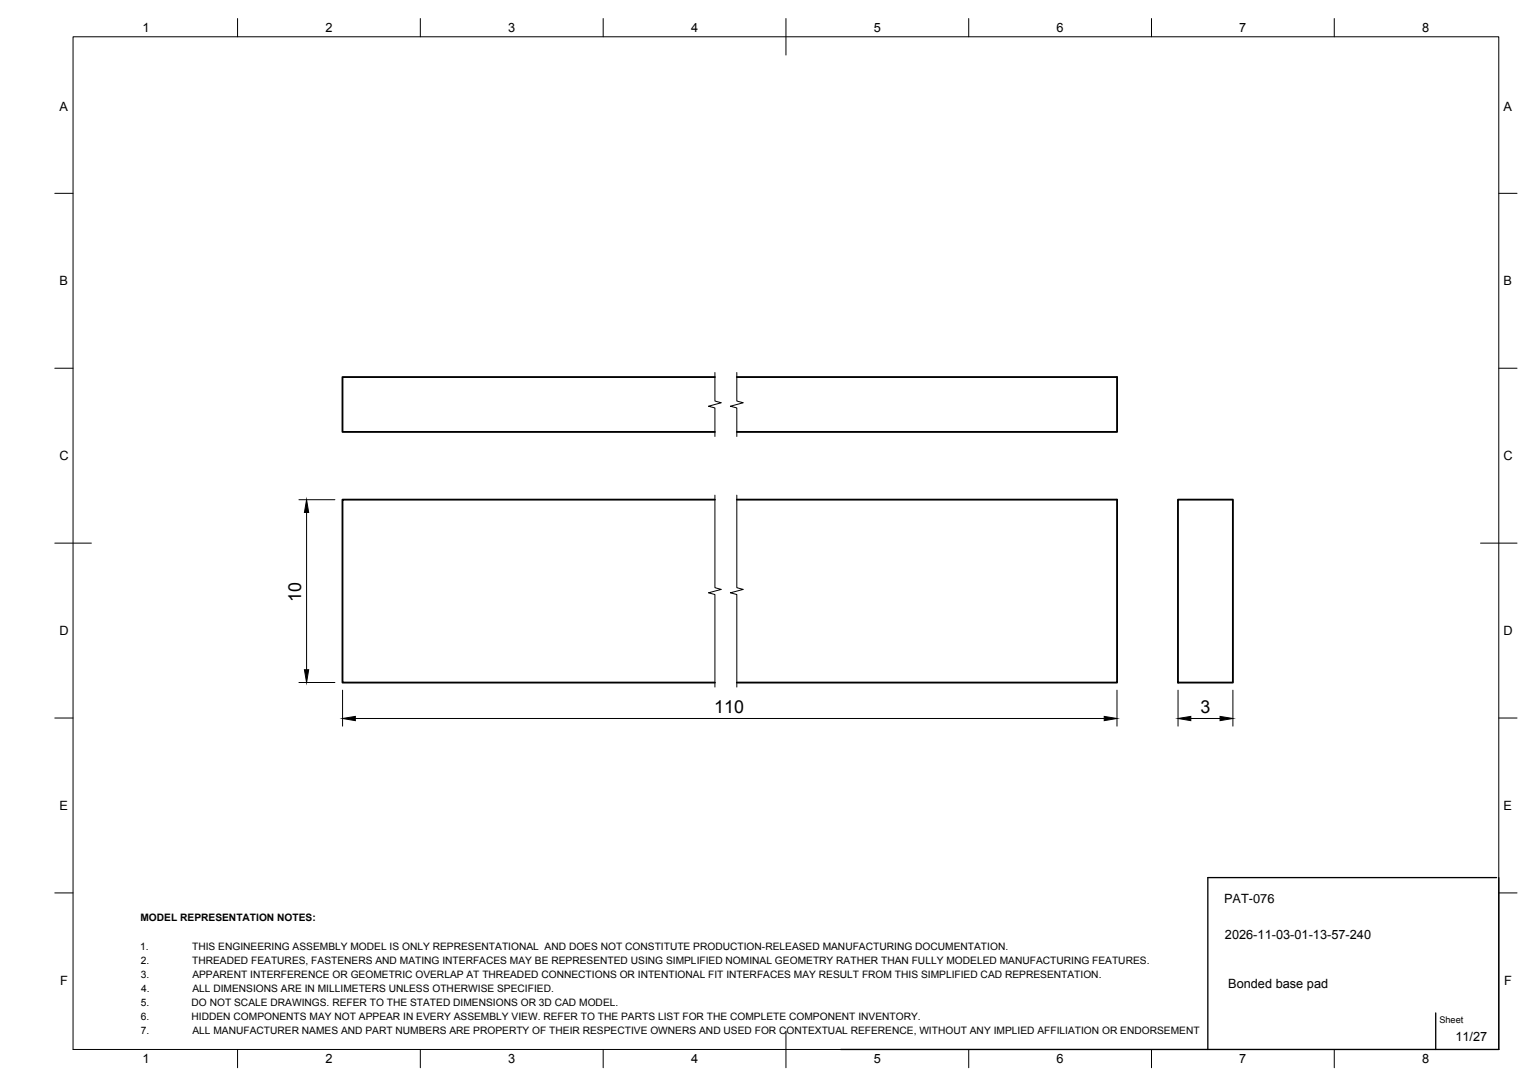
ISO-10303-21;
HEADER;
/* Generated by software containing ST-Developer
 * from STEP Tools, Inc. (www.steptools.com) 
 */

FILE_DESCRIPTION(
/* description */ ('Overhung pulley bearing cartridge'),
/* implementation_level */ '2;1');

FILE_NAME(
/* name */ 'Bonded base pad.step',
/* time_stamp */ '2026-10-28T03:22:33-07:00',
/* author */ (''),
/* organization */ (''),
/* preprocessor_version */ 'ST-DEVELOPER v20.2',
/* originating_system */ 'Autodesk Translation Framework v15.17.0.0',
/* authorisation */ '');

FILE_SCHEMA (('AUTOMOTIVE_DESIGN { 1 0 10303 214 3 1 1 }'));
ENDSEC;

DATA;
#10=MECHANICAL_DESIGN_GEOMETRIC_PRESENTATION_REPRESENTATION('',(#289),#10963);
#245=SHAPE_REPRESENTATION_RELATIONSHIP('SRR','None',#11065,#267);
#267=ADVANCED_BREP_SHAPE_REPRESENTATION('',(#319),#10945);
#289=STYLED_ITEM('',(#11232),#319);
#319=MANIFOLD_SOLID_BREP('Body1',#5656);
#479=PLANE('',#6098);
#480=PLANE('',#6099);
#481=PLANE('',#6100);
#482=PLANE('',#6101);
#483=PLANE('',#6102);
#484=PLANE('',#6103);
#659=FACE_OUTER_BOUND('',#1043,.T.);
#660=FACE_OUTER_BOUND('',#1044,.T.);
#661=FACE_OUTER_BOUND('',#1045,.T.);
#662=FACE_OUTER_BOUND('',#1046,.T.);
#663=FACE_OUTER_BOUND('',#1047,.T.);
#664=FACE_OUTER_BOUND('',#1048,.T.);
#1043=EDGE_LOOP('',(#3987,#3988,#3989,#3990));
#1044=EDGE_LOOP('',(#3991,#3992,#3993,#3994));
#1045=EDGE_LOOP('',(#3995,#3996,#3997,#3998));
#1046=EDGE_LOOP('',(#3999,#4000,#4001,#4002));
#1047=EDGE_LOOP('',(#4003,#4004,#4005,#4006));
#1048=EDGE_LOOP('',(#4007,#4008,#4009,#4010));
#1413=LINE('',#8927,#1755);
#1414=LINE('',#8929,#1756);
#1415=LINE('',#8931,#1757);
#1416=LINE('',#8932,#1758);
#1417=LINE('',#8935,#1759);
#1418=LINE('',#8937,#1760);
#1419=LINE('',#8938,#1761);
#1420=LINE('',#8941,#1762);
#1421=LINE('',#8943,#1763);
#1422=LINE('',#8944,#1764);
#1423=LINE('',#8946,#1765);
#1424=LINE('',#8947,#1766);
#1755=VECTOR('',#7121,1.);
#1756=VECTOR('',#7122,1.);
#1757=VECTOR('',#7123,1.);
#1758=VECTOR('',#7124,1.);
#1759=VECTOR('',#7127,1.);
#1760=VECTOR('',#7128,1.);
#1761=VECTOR('',#7129,1.);
#1762=VECTOR('',#7132,1.);
#1763=VECTOR('',#7133,1.);
#1764=VECTOR('',#7134,1.);
#1765=VECTOR('',#7137,1.);
#1766=VECTOR('',#7138,1.);
#2493=VERTEX_POINT('',#8925);
#2494=VERTEX_POINT('',#8926);
#2495=VERTEX_POINT('',#8928);
#2496=VERTEX_POINT('',#8930);
#2497=VERTEX_POINT('',#8934);
#2498=VERTEX_POINT('',#8936);
#2499=VERTEX_POINT('',#8940);
#2500=VERTEX_POINT('',#8942);
#3063=EDGE_CURVE('',#2493,#2494,#1413,.T.);
#3064=EDGE_CURVE('',#2494,#2495,#1414,.T.);
#3065=EDGE_CURVE('',#2496,#2495,#1415,.T.);
#3066=EDGE_CURVE('',#2493,#2496,#1416,.T.);
#3067=EDGE_CURVE('',#2497,#2493,#1417,.T.);
#3068=EDGE_CURVE('',#2498,#2496,#1418,.T.);
#3069=EDGE_CURVE('',#2497,#2498,#1419,.T.);
#3070=EDGE_CURVE('',#2499,#2497,#1420,.T.);
#3071=EDGE_CURVE('',#2500,#2498,#1421,.T.);
#3072=EDGE_CURVE('',#2499,#2500,#1422,.T.);
#3073=EDGE_CURVE('',#2494,#2499,#1423,.T.);
#3074=EDGE_CURVE('',#2495,#2500,#1424,.T.);
#3987=ORIENTED_EDGE('',*,*,#3063,.T.);
#3988=ORIENTED_EDGE('',*,*,#3064,.T.);
#3989=ORIENTED_EDGE('',*,*,#3065,.F.);
#3990=ORIENTED_EDGE('',*,*,#3066,.F.);
#3991=ORIENTED_EDGE('',*,*,#3067,.T.);
#3992=ORIENTED_EDGE('',*,*,#3066,.T.);
#3993=ORIENTED_EDGE('',*,*,#3068,.F.);
#3994=ORIENTED_EDGE('',*,*,#3069,.F.);
#3995=ORIENTED_EDGE('',*,*,#3070,.T.);
#3996=ORIENTED_EDGE('',*,*,#3069,.T.);
#3997=ORIENTED_EDGE('',*,*,#3071,.F.);
#3998=ORIENTED_EDGE('',*,*,#3072,.F.);
#3999=ORIENTED_EDGE('',*,*,#3073,.T.);
#4000=ORIENTED_EDGE('',*,*,#3072,.T.);
#4001=ORIENTED_EDGE('',*,*,#3074,.F.);
#4002=ORIENTED_EDGE('',*,*,#3064,.F.);
#4003=ORIENTED_EDGE('',*,*,#3074,.T.);
#4004=ORIENTED_EDGE('',*,*,#3071,.T.);
#4005=ORIENTED_EDGE('',*,*,#3068,.T.);
#4006=ORIENTED_EDGE('',*,*,#3065,.T.);
#4007=ORIENTED_EDGE('',*,*,#3073,.F.);
#4008=ORIENTED_EDGE('',*,*,#3063,.F.);
#4009=ORIENTED_EDGE('',*,*,#3067,.F.);
#4010=ORIENTED_EDGE('',*,*,#3070,.F.);
#5403=ADVANCED_FACE('',(#659),#479,.T.);
#5404=ADVANCED_FACE('',(#660),#480,.T.);
#5405=ADVANCED_FACE('',(#661),#481,.T.);
#5406=ADVANCED_FACE('',(#662),#482,.T.);
#5407=ADVANCED_FACE('',(#663),#483,.T.);
#5408=ADVANCED_FACE('',(#664),#484,.F.);
#5656=CLOSED_SHELL('',(#5403,#5404,#5405,#5406,#5407,#5408));
#6097=AXIS2_PLACEMENT_3D('',#8923,#7117,#7118);
#6098=AXIS2_PLACEMENT_3D('',#8924,#7119,#7120);
#6099=AXIS2_PLACEMENT_3D('',#8933,#7125,#7126);
#6100=AXIS2_PLACEMENT_3D('',#8939,#7130,#7131);
#6101=AXIS2_PLACEMENT_3D('',#8945,#7135,#7136);
#6102=AXIS2_PLACEMENT_3D('',#8948,#7139,#7140);
#6103=AXIS2_PLACEMENT_3D('',#8949,#7141,#7142);
#7117=DIRECTION('axis',(0.,0.,1.));
#7118=DIRECTION('refdir',(1.,0.,0.));
#7119=DIRECTION('center_axis',(0.,1.,0.));
#7120=DIRECTION('ref_axis',(-1.,0.,0.));
#7121=DIRECTION('',(-1.,0.,0.));
#7122=DIRECTION('',(0.,0.,1.));
#7123=DIRECTION('',(-1.,0.,0.));
#7124=DIRECTION('',(0.,0.,1.));
#7125=DIRECTION('center_axis',(1.,0.,0.));
#7126=DIRECTION('ref_axis',(0.,1.,0.));
#7127=DIRECTION('',(0.,1.,0.));
#7128=DIRECTION('',(0.,1.,0.));
#7129=DIRECTION('',(0.,0.,1.));
#7130=DIRECTION('center_axis',(0.,-1.,0.));
#7131=DIRECTION('ref_axis',(1.,0.,0.));
#7132=DIRECTION('',(1.,0.,0.));
#7133=DIRECTION('',(1.,0.,0.));
#7134=DIRECTION('',(0.,0.,1.));
#7135=DIRECTION('center_axis',(-1.,0.,0.));
#7136=DIRECTION('ref_axis',(0.,-1.,0.));
#7137=DIRECTION('',(0.,-1.,0.));
#7138=DIRECTION('',(0.,-1.,0.));
#7139=DIRECTION('center_axis',(0.,0.,1.));
#7140=DIRECTION('ref_axis',(1.,0.,0.));
#7141=DIRECTION('center_axis',(0.,0.,1.));
#7142=DIRECTION('ref_axis',(1.,0.,0.));
#8923=CARTESIAN_POINT('',(0.,0.,0.));
#8924=CARTESIAN_POINT('Origin',(5.5,0.,-0.3));
#8925=CARTESIAN_POINT('',(5.5,0.,-0.3));
#8926=CARTESIAN_POINT('',(-5.5,0.,-0.3));
#8927=CARTESIAN_POINT('',(5.5,0.,-0.3));
#8928=CARTESIAN_POINT('',(-5.5,0.,0.));
#8929=CARTESIAN_POINT('',(-5.5,0.,-0.3));
#8930=CARTESIAN_POINT('',(5.5,0.,0.));
#8931=CARTESIAN_POINT('',(5.5,0.,0.));
#8932=CARTESIAN_POINT('',(5.5,0.,-0.3));
#8933=CARTESIAN_POINT('Origin',(5.5,-1.,-0.3));
#8934=CARTESIAN_POINT('',(5.5,-1.,-0.3));
#8935=CARTESIAN_POINT('',(5.5,-1.,-0.3));
#8936=CARTESIAN_POINT('',(5.5,-1.,0.));
#8937=CARTESIAN_POINT('',(5.5,-1.,0.));
#8938=CARTESIAN_POINT('',(5.5,-1.,-0.3));
#8939=CARTESIAN_POINT('Origin',(-5.5,-1.,-0.3));
#8940=CARTESIAN_POINT('',(-5.5,-1.,-0.3));
#8941=CARTESIAN_POINT('',(-5.5,-1.,-0.3));
#8942=CARTESIAN_POINT('',(-5.5,-1.,0.));
#8943=CARTESIAN_POINT('',(-5.5,-1.,0.));
#8944=CARTESIAN_POINT('',(-5.5,-1.,-0.3));
#8945=CARTESIAN_POINT('Origin',(-5.5,0.,-0.3));
#8946=CARTESIAN_POINT('',(-5.5,0.,-0.3));
#8947=CARTESIAN_POINT('',(-5.5,0.,0.));
#8948=CARTESIAN_POINT('Origin',(0.,-0.5,0.));
#8949=CARTESIAN_POINT('Origin',(0.,-0.5,-0.3));
#10918=UNCERTAINTY_MEASURE_WITH_UNIT(LENGTH_MEASURE(0.001),#10964,
'DISTANCE_ACCURACY_VALUE',
'Maximum model space distance between geometric entities at asserted c
onnectivities');
#10936=UNCERTAINTY_MEASURE_WITH_UNIT(LENGTH_MEASURE(0.001),#10964,
'DISTANCE_ACCURACY_VALUE',
'Maximum model space distance between geometric entities at asserted c
onnectivities');
#10945=(
GEOMETRIC_REPRESENTATION_CONTEXT(3)
GLOBAL_UNCERTAINTY_ASSIGNED_CONTEXT((#10918))
GLOBAL_UNIT_ASSIGNED_CONTEXT((#10964,#10966,#10967))
REPRESENTATION_CONTEXT('','3D')
);
#10963=(
GEOMETRIC_REPRESENTATION_CONTEXT(3)
GLOBAL_UNCERTAINTY_ASSIGNED_CONTEXT((#10936))
GLOBAL_UNIT_ASSIGNED_CONTEXT((#10964,#10966,#10967))
REPRESENTATION_CONTEXT('','3D')
);
#10964=(
LENGTH_UNIT()
NAMED_UNIT(*)
SI_UNIT(.CENTI.,.METRE.)
);
#10966=(
NAMED_UNIT(*)
PLANE_ANGLE_UNIT()
SI_UNIT($,.RADIAN.)
);
#10967=(
NAMED_UNIT(*)
SI_UNIT($,.STERADIAN.)
SOLID_ANGLE_UNIT()
);
#10976=SHAPE_DEFINITION_REPRESENTATION(#11002,#11065);
#11002=PRODUCT_DEFINITION_SHAPE('',$,#11092);
#11065=SHAPE_REPRESENTATION('',(#6097),#10945);
#11083=PRODUCT_DEFINITION_CONTEXT('part definition',#11163,'design');
#11092=PRODUCT_DEFINITION('Bonded base pad','Bonded base pad',#11118,#11083);
#11118=PRODUCT_DEFINITION_FORMATION('',$,#11173);
#11163=APPLICATION_CONTEXT(
'Core Data for Automotive Mechanical Design Process');
#11164=PRODUCT_CONTEXT('part definition',#11163,'mechanical');
#11173=PRODUCT('Bonded base pad','Bonded base pad','Bonded base pad',(#11164));
#11226=COLOUR_RGB('Dark Blue',0.08,0.2,0.34);
#11227=FILL_AREA_STYLE_COLOUR('',#11226);
#11228=FILL_AREA_STYLE('',(#11227));
#11229=SURFACE_STYLE_FILL_AREA(#11228);
#11230=SURFACE_SIDE_STYLE('',(#11229));
#11231=SURFACE_STYLE_USAGE(.BOTH.,#11230);
#11232=PRESENTATION_STYLE_ASSIGNMENT((#11231));
ENDSEC;
END-ISO-10303-21;
